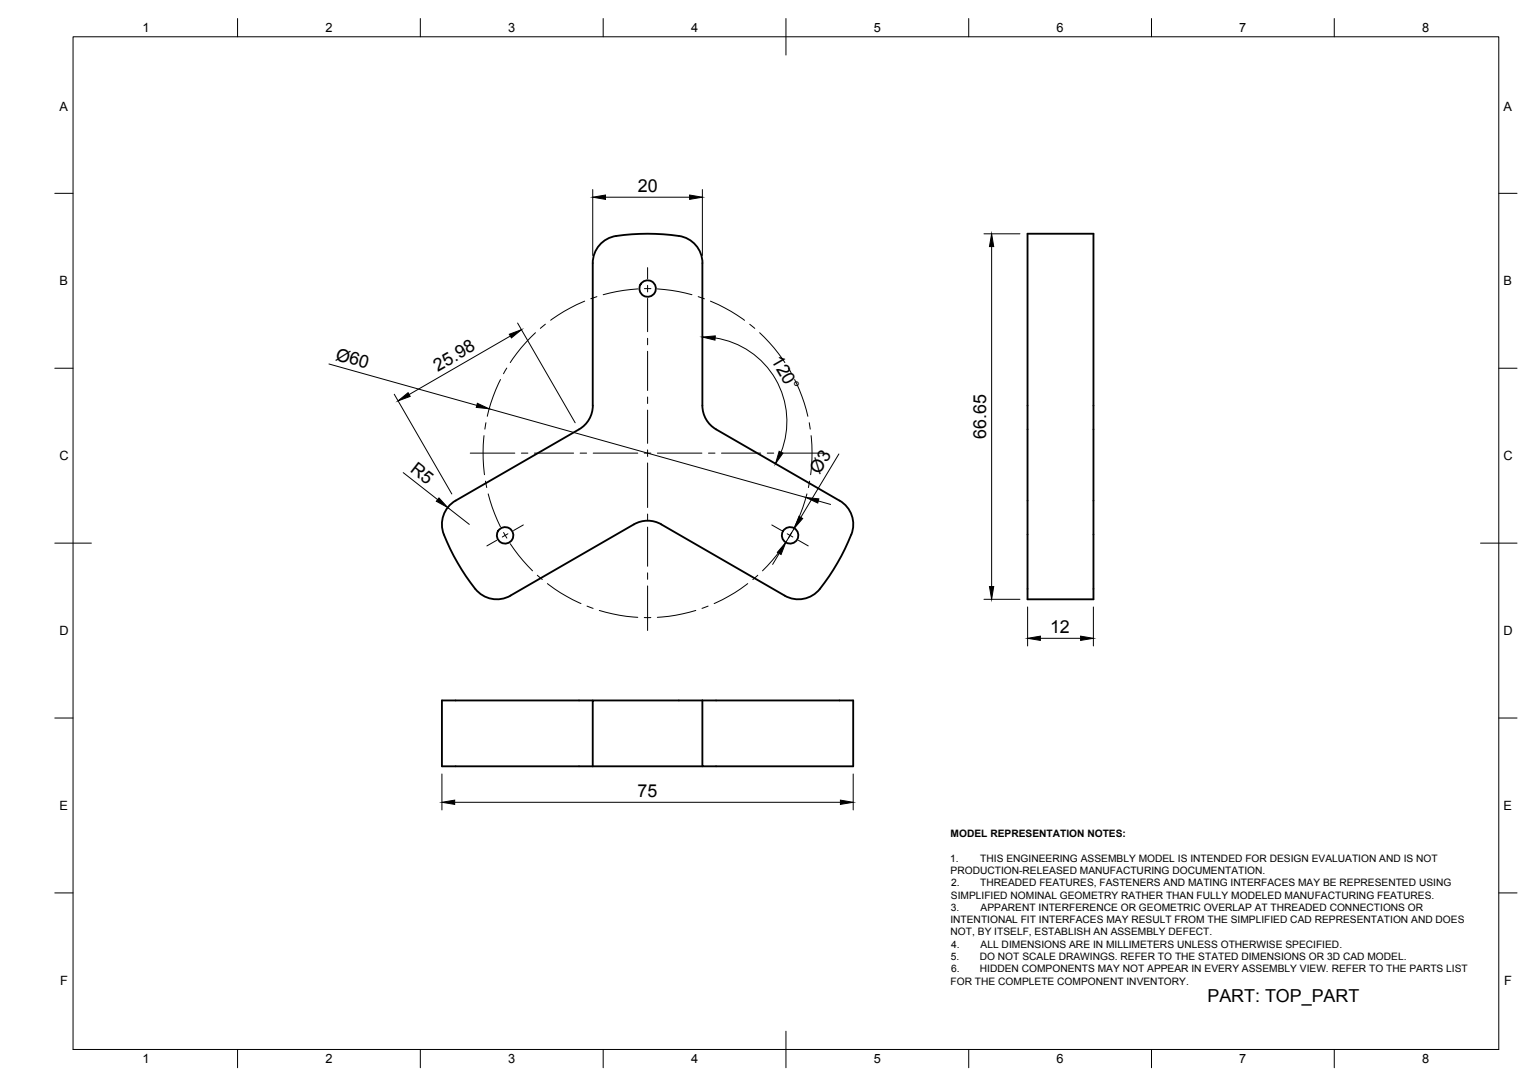
ISO-10303-21;
HEADER;
/* Generated by software containing ST-Developer
 * from STEP Tools, Inc. (www.steptools.com) 
 */

FILE_DESCRIPTION(
/* description */ (''),
/* implementation_level */ '2;1');

FILE_NAME(
/* name */ 'Top_Part.step',
/* time_stamp */ '2026-10-05T00:14:20-07:00',
/* author */ (''),
/* organization */ (''),
/* preprocessor_version */ 'ST-DEVELOPER v20.2',
/* originating_system */ 'Autodesk Translation Framework v15.15.0.0',
/* authorisation */ '');

FILE_SCHEMA (('AUTOMOTIVE_DESIGN { 1 0 10303 214 3 1 1 }'));
ENDSEC;

DATA;
#10=MECHANICAL_DESIGN_GEOMETRIC_PRESENTATION_REPRESENTATION('',(#3375),#75336);
#3359=SHAPE_REPRESENTATION_RELATIONSHIP('SRR','None',#75372,#3367);
#3367=ADVANCED_BREP_SHAPE_REPRESENTATION('',(#3383),#75332);
#3375=STYLED_ITEM('',(#75417),#3383);
#3383=MANIFOLD_SOLID_BREP('Body1',#32025);
#3388=FACE_BOUND('',#6889,.T.);
#3389=FACE_BOUND('',#6890,.T.);
#3390=FACE_BOUND('',#6891,.T.);
#3391=FACE_BOUND('',#6903,.T.);
#3392=FACE_BOUND('',#6904,.T.);
#3393=FACE_BOUND('',#6905,.T.);
#3405=CIRCLE('',#32145,1.5);
#3406=CIRCLE('',#32146,1.5);
#3407=CIRCLE('',#32148,1.5);
#3408=CIRCLE('',#32149,1.5);
#3409=CIRCLE('',#32151,1.5);
#3410=CIRCLE('',#32152,1.5);
#3411=CIRCLE('',#32154,5.);
#3412=CIRCLE('',#32155,5.);
#3413=CIRCLE('',#32158,5.);
#3414=CIRCLE('',#32159,5.);
#3415=CIRCLE('',#32162,5.);
#3416=CIRCLE('',#32163,5.);
#3417=CIRCLE('',#32166,5.);
#3418=CIRCLE('',#32167,5.);
#3419=CIRCLE('',#32169,40.);
#3420=CIRCLE('',#32170,40.);
#3421=CIRCLE('',#32172,5.);
#3422=CIRCLE('',#32173,40.);
#3423=CIRCLE('',#32174,5.);
#3424=CIRCLE('',#32175,5.);
#3425=CIRCLE('',#32176,40.);
#3426=CIRCLE('',#32177,5.);
#3427=CIRCLE('',#32178,5.);
#3428=CIRCLE('',#32180,5.);
#3429=CIRCLE('',#32182,40.);
#3430=CIRCLE('',#32184,5.);
#3431=CIRCLE('',#32186,5.);
#3432=CIRCLE('',#32188,5.);
#3433=CIRCLE('',#32190,5.);
#3434=CIRCLE('',#32193,40.);
#4456=CYLINDRICAL_SURFACE('',#32144,1.5);
#4457=CYLINDRICAL_SURFACE('',#32147,1.5);
#4458=CYLINDRICAL_SURFACE('',#32150,1.5);
#4459=CYLINDRICAL_SURFACE('',#32153,5.);
#4460=CYLINDRICAL_SURFACE('',#32157,5.);
#4461=CYLINDRICAL_SURFACE('',#32161,5.);
#4462=CYLINDRICAL_SURFACE('',#32165,5.);
#4463=CYLINDRICAL_SURFACE('',#32168,40.);
#4464=CYLINDRICAL_SURFACE('',#32179,5.);
#4465=CYLINDRICAL_SURFACE('',#32181,40.);
#4466=CYLINDRICAL_SURFACE('',#32183,5.);
#4467=CYLINDRICAL_SURFACE('',#32185,5.);
#4468=CYLINDRICAL_SURFACE('',#32187,5.);
#4469=CYLINDRICAL_SURFACE('',#32189,5.);
#4470=CYLINDRICAL_SURFACE('',#32192,40.);
#5149=FACE_OUTER_BOUND('',#6877,.T.);
#5150=FACE_OUTER_BOUND('',#6878,.T.);
#5151=FACE_OUTER_BOUND('',#6879,.T.);
#5152=FACE_OUTER_BOUND('',#6880,.T.);
#5153=FACE_OUTER_BOUND('',#6881,.T.);
#5154=FACE_OUTER_BOUND('',#6882,.T.);
#5155=FACE_OUTER_BOUND('',#6883,.T.);
#5156=FACE_OUTER_BOUND('',#6884,.T.);
#5157=FACE_OUTER_BOUND('',#6885,.T.);
#5158=FACE_OUTER_BOUND('',#6886,.T.);
#5159=FACE_OUTER_BOUND('',#6887,.T.);
#5160=FACE_OUTER_BOUND('',#6888,.T.);
#5161=FACE_OUTER_BOUND('',#6892,.T.);
#5162=FACE_OUTER_BOUND('',#6893,.T.);
#5163=FACE_OUTER_BOUND('',#6894,.T.);
#5164=FACE_OUTER_BOUND('',#6895,.T.);
#5165=FACE_OUTER_BOUND('',#6896,.T.);
#5166=FACE_OUTER_BOUND('',#6897,.T.);
#5167=FACE_OUTER_BOUND('',#6898,.T.);
#5168=FACE_OUTER_BOUND('',#6899,.T.);
#5169=FACE_OUTER_BOUND('',#6900,.T.);
#5170=FACE_OUTER_BOUND('',#6901,.T.);
#5171=FACE_OUTER_BOUND('',#6902,.T.);
#6877=EDGE_LOOP('',(#19631,#19632,#19633,#19634));
#6878=EDGE_LOOP('',(#19635,#19636,#19637,#19638));
#6879=EDGE_LOOP('',(#19639,#19640,#19641,#19642));
#6880=EDGE_LOOP('',(#19643,#19644,#19645,#19646));
#6881=EDGE_LOOP('',(#19647,#19648,#19649,#19650));
#6882=EDGE_LOOP('',(#19651,#19652,#19653,#19654));
#6883=EDGE_LOOP('',(#19655,#19656,#19657,#19658));
#6884=EDGE_LOOP('',(#19659,#19660,#19661,#19662));
#6885=EDGE_LOOP('',(#19663,#19664,#19665,#19666));
#6886=EDGE_LOOP('',(#19667,#19668,#19669,#19670));
#6887=EDGE_LOOP('',(#19671,#19672,#19673,#19674));
#6888=EDGE_LOOP('',(#19675,#19676,#19677,#19678,#19679,#19680,#19681,#19682,
#19683,#19684,#19685,#19686,#19687,#19688,#19689,#19690,#19691,#19692));
#6889=EDGE_LOOP('',(#19693));
#6890=EDGE_LOOP('',(#19694));
#6891=EDGE_LOOP('',(#19695));
#6892=EDGE_LOOP('',(#19696,#19697,#19698,#19699));
#6893=EDGE_LOOP('',(#19700,#19701,#19702,#19703));
#6894=EDGE_LOOP('',(#19704,#19705,#19706,#19707));
#6895=EDGE_LOOP('',(#19708,#19709,#19710,#19711));
#6896=EDGE_LOOP('',(#19712,#19713,#19714,#19715));
#6897=EDGE_LOOP('',(#19716,#19717,#19718,#19719));
#6898=EDGE_LOOP('',(#19720,#19721,#19722,#19723));
#6899=EDGE_LOOP('',(#19724,#19725,#19726,#19727));
#6900=EDGE_LOOP('',(#19728,#19729,#19730,#19731));
#6901=EDGE_LOOP('',(#19732,#19733,#19734,#19735));
#6902=EDGE_LOOP('',(#19736,#19737,#19738,#19739,#19740,#19741,#19742,#19743,
#19744,#19745,#19746,#19747,#19748,#19749,#19750,#19751,#19752,#19753));
#6903=EDGE_LOOP('',(#19754));
#6904=EDGE_LOOP('',(#19755));
#6905=EDGE_LOOP('',(#19756));
#8623=LINE('',#46118,#9869);
#8624=LINE('',#46124,#9870);
#8625=LINE('',#46130,#9871);
#8626=LINE('',#46137,#9872);
#8627=LINE('',#46140,#9873);
#8628=LINE('',#46143,#9874);
#8629=LINE('',#46145,#9875);
#8630=LINE('',#46146,#9876);
#8631=LINE('',#46152,#9877);
#8632=LINE('',#46155,#9878);
#8633=LINE('',#46158,#9879);
#8634=LINE('',#46160,#9880);
#8635=LINE('',#46161,#9881);
#8636=LINE('',#46167,#9882);
#8637=LINE('',#46170,#9883);
#8638=LINE('',#46173,#9884);
#8639=LINE('',#46175,#9885);
#8640=LINE('',#46176,#9886);
#8641=LINE('',#46182,#9887);
#8642=LINE('',#46185,#9888);
#8643=LINE('',#46190,#9889);
#8644=LINE('',#46193,#9890);
#8645=LINE('',#46200,#9891);
#8646=LINE('',#46207,#9892);
#8647=LINE('',#46212,#9893);
#8648=LINE('',#46216,#9894);
#8649=LINE('',#46220,#9895);
#8650=LINE('',#46224,#9896);
#8651=LINE('',#46229,#9897);
#8652=LINE('',#46232,#9898);
#8653=LINE('',#46234,#9899);
#8654=LINE('',#46238,#9900);
#8655=LINE('',#46240,#9901);
#9869=VECTOR('',#36423,1.5);
#9870=VECTOR('',#36430,1.5);
#9871=VECTOR('',#36437,1.5);
#9872=VECTOR('',#36444,10.);
#9873=VECTOR('',#36447,10.);
#9874=VECTOR('',#36450,10.);
#9875=VECTOR('',#36451,10.);
#9876=VECTOR('',#36452,10.);
#9877=VECTOR('',#36457,10.);
#9878=VECTOR('',#36460,10.);
#9879=VECTOR('',#36463,10.);
#9880=VECTOR('',#36464,10.);
#9881=VECTOR('',#36465,10.);
#9882=VECTOR('',#36470,10.);
#9883=VECTOR('',#36473,10.);
#9884=VECTOR('',#36476,9.99999999999999);
#9885=VECTOR('',#36477,10.);
#9886=VECTOR('',#36478,9.99999999999999);
#9887=VECTOR('',#36483,10.);
#9888=VECTOR('',#36486,10.);
#9889=VECTOR('',#36491,10.);
#9890=VECTOR('',#36496,9.99999999999999);
#9891=VECTOR('',#36503,10.);
#9892=VECTOR('',#36510,10.);
#9893=VECTOR('',#36517,10.);
#9894=VECTOR('',#36522,10.);
#9895=VECTOR('',#36527,10.);
#9896=VECTOR('',#36532,10.);
#9897=VECTOR('',#36539,10.);
#9898=VECTOR('',#36542,10.);
#9899=VECTOR('',#36545,10.);
#9900=VECTOR('',#36552,10.);
#9901=VECTOR('',#36555,9.99999999999999);
#11114=VERTEX_POINT('',#46115);
#11115=VERTEX_POINT('',#46117);
#11116=VERTEX_POINT('',#46121);
#11117=VERTEX_POINT('',#46123);
#11118=VERTEX_POINT('',#46127);
#11119=VERTEX_POINT('',#46129);
#11120=VERTEX_POINT('',#46133);
#11121=VERTEX_POINT('',#46134);
#11122=VERTEX_POINT('',#46136);
#11123=VERTEX_POINT('',#46138);
#11124=VERTEX_POINT('',#46142);
#11125=VERTEX_POINT('',#46144);
#11126=VERTEX_POINT('',#46148);
#11127=VERTEX_POINT('',#46149);
#11128=VERTEX_POINT('',#46151);
#11129=VERTEX_POINT('',#46153);
#11130=VERTEX_POINT('',#46157);
#11131=VERTEX_POINT('',#46159);
#11132=VERTEX_POINT('',#46163);
#11133=VERTEX_POINT('',#46164);
#11134=VERTEX_POINT('',#46166);
#11135=VERTEX_POINT('',#46168);
#11136=VERTEX_POINT('',#46172);
#11137=VERTEX_POINT('',#46174);
#11138=VERTEX_POINT('',#46178);
#11139=VERTEX_POINT('',#46179);
#11140=VERTEX_POINT('',#46181);
#11141=VERTEX_POINT('',#46183);
#11142=VERTEX_POINT('',#46187);
#11143=VERTEX_POINT('',#46189);
#11144=VERTEX_POINT('',#46194);
#11145=VERTEX_POINT('',#46196);
#11146=VERTEX_POINT('',#46198);
#11147=VERTEX_POINT('',#46201);
#11148=VERTEX_POINT('',#46203);
#11149=VERTEX_POINT('',#46205);
#11150=VERTEX_POINT('',#46210);
#11151=VERTEX_POINT('',#46214);
#11152=VERTEX_POINT('',#46218);
#11153=VERTEX_POINT('',#46222);
#11154=VERTEX_POINT('',#46228);
#11155=VERTEX_POINT('',#46230);
#14510=EDGE_CURVE('',#11114,#11114,#3405,.T.);
#14511=EDGE_CURVE('',#11114,#11115,#8623,.T.);
#14512=EDGE_CURVE('',#11115,#11115,#3406,.T.);
#14513=EDGE_CURVE('',#11116,#11116,#3407,.T.);
#14514=EDGE_CURVE('',#11116,#11117,#8624,.T.);
#14515=EDGE_CURVE('',#11117,#11117,#3408,.T.);
#14516=EDGE_CURVE('',#11118,#11118,#3409,.T.);
#14517=EDGE_CURVE('',#11118,#11119,#8625,.T.);
#14518=EDGE_CURVE('',#11119,#11119,#3410,.T.);
#14519=EDGE_CURVE('',#11120,#11121,#3411,.T.);
#14520=EDGE_CURVE('',#11121,#11122,#8626,.T.);
#14521=EDGE_CURVE('',#11122,#11123,#3412,.T.);
#14522=EDGE_CURVE('',#11123,#11120,#8627,.T.);
#14523=EDGE_CURVE('',#11121,#11124,#8628,.T.);
#14524=EDGE_CURVE('',#11125,#11124,#8629,.T.);
#14525=EDGE_CURVE('',#11122,#11125,#8630,.T.);
#14526=EDGE_CURVE('',#11126,#11127,#3413,.T.);
#14527=EDGE_CURVE('',#11127,#11128,#8631,.T.);
#14528=EDGE_CURVE('',#11128,#11129,#3414,.T.);
#14529=EDGE_CURVE('',#11129,#11126,#8632,.T.);
#14530=EDGE_CURVE('',#11127,#11130,#8633,.T.);
#14531=EDGE_CURVE('',#11131,#11130,#8634,.T.);
#14532=EDGE_CURVE('',#11128,#11131,#8635,.T.);
#14533=EDGE_CURVE('',#11132,#11133,#3415,.T.);
#14534=EDGE_CURVE('',#11133,#11134,#8636,.T.);
#14535=EDGE_CURVE('',#11134,#11135,#3416,.T.);
#14536=EDGE_CURVE('',#11135,#11132,#8637,.T.);
#14537=EDGE_CURVE('',#11133,#11136,#8638,.T.);
#14538=EDGE_CURVE('',#11137,#11136,#8639,.T.);
#14539=EDGE_CURVE('',#11134,#11137,#8640,.T.);
#14540=EDGE_CURVE('',#11138,#11139,#3417,.T.);
#14541=EDGE_CURVE('',#11139,#11140,#8641,.T.);
#14542=EDGE_CURVE('',#11140,#11141,#3418,.T.);
#14543=EDGE_CURVE('',#11141,#11138,#8642,.T.);
#14544=EDGE_CURVE('',#11142,#11139,#3419,.T.);
#14545=EDGE_CURVE('',#11143,#11142,#8643,.T.);
#14546=EDGE_CURVE('',#11143,#11140,#3420,.T.);
#14547=EDGE_CURVE('',#11138,#11129,#8644,.T.);
#14548=EDGE_CURVE('',#11144,#11131,#3421,.T.);
#14549=EDGE_CURVE('',#11144,#11145,#3422,.T.);
#14550=EDGE_CURVE('',#11146,#11145,#3423,.T.);
#14551=EDGE_CURVE('',#11146,#11123,#8645,.T.);
#14552=EDGE_CURVE('',#11147,#11125,#3424,.T.);
#14553=EDGE_CURVE('',#11147,#11148,#3425,.T.);
#14554=EDGE_CURVE('',#11149,#11148,#3426,.T.);
#14555=EDGE_CURVE('',#11149,#11135,#8646,.T.);
#14556=EDGE_CURVE('',#11142,#11137,#3427,.T.);
#14557=EDGE_CURVE('',#11130,#11150,#3428,.T.);
#14558=EDGE_CURVE('',#11150,#11144,#8647,.T.);
#14559=EDGE_CURVE('',#11150,#11151,#3429,.T.);
#14560=EDGE_CURVE('',#11145,#11151,#8648,.T.);
#14561=EDGE_CURVE('',#11151,#11152,#3430,.T.);
#14562=EDGE_CURVE('',#11152,#11146,#8649,.T.);
#14563=EDGE_CURVE('',#11124,#11153,#3431,.T.);
#14564=EDGE_CURVE('',#11153,#11147,#8650,.T.);
#14565=EDGE_CURVE('',#11136,#11143,#3432,.T.);
#14566=EDGE_CURVE('',#11148,#11154,#8651,.T.);
#14567=EDGE_CURVE('',#11154,#11155,#3433,.T.);
#14568=EDGE_CURVE('',#11155,#11149,#8652,.T.);
#14569=EDGE_CURVE('',#11155,#11132,#8653,.T.);
#14570=EDGE_CURVE('',#11153,#11154,#3434,.T.);
#14571=EDGE_CURVE('',#11152,#11120,#8654,.T.);
#14572=EDGE_CURVE('',#11141,#11126,#8655,.T.);
#19631=ORIENTED_EDGE('',*,*,#14510,.F.);
#19632=ORIENTED_EDGE('',*,*,#14511,.T.);
#19633=ORIENTED_EDGE('',*,*,#14512,.F.);
#19634=ORIENTED_EDGE('',*,*,#14511,.F.);
#19635=ORIENTED_EDGE('',*,*,#14513,.F.);
#19636=ORIENTED_EDGE('',*,*,#14514,.T.);
#19637=ORIENTED_EDGE('',*,*,#14515,.F.);
#19638=ORIENTED_EDGE('',*,*,#14514,.F.);
#19639=ORIENTED_EDGE('',*,*,#14516,.F.);
#19640=ORIENTED_EDGE('',*,*,#14517,.T.);
#19641=ORIENTED_EDGE('',*,*,#14518,.F.);
#19642=ORIENTED_EDGE('',*,*,#14517,.F.);
#19643=ORIENTED_EDGE('',*,*,#14519,.T.);
#19644=ORIENTED_EDGE('',*,*,#14520,.T.);
#19645=ORIENTED_EDGE('',*,*,#14521,.T.);
#19646=ORIENTED_EDGE('',*,*,#14522,.T.);
#19647=ORIENTED_EDGE('',*,*,#14520,.F.);
#19648=ORIENTED_EDGE('',*,*,#14523,.T.);
#19649=ORIENTED_EDGE('',*,*,#14524,.F.);
#19650=ORIENTED_EDGE('',*,*,#14525,.F.);
#19651=ORIENTED_EDGE('',*,*,#14526,.T.);
#19652=ORIENTED_EDGE('',*,*,#14527,.T.);
#19653=ORIENTED_EDGE('',*,*,#14528,.T.);
#19654=ORIENTED_EDGE('',*,*,#14529,.T.);
#19655=ORIENTED_EDGE('',*,*,#14527,.F.);
#19656=ORIENTED_EDGE('',*,*,#14530,.T.);
#19657=ORIENTED_EDGE('',*,*,#14531,.F.);
#19658=ORIENTED_EDGE('',*,*,#14532,.F.);
#19659=ORIENTED_EDGE('',*,*,#14533,.T.);
#19660=ORIENTED_EDGE('',*,*,#14534,.T.);
#19661=ORIENTED_EDGE('',*,*,#14535,.T.);
#19662=ORIENTED_EDGE('',*,*,#14536,.T.);
#19663=ORIENTED_EDGE('',*,*,#14534,.F.);
#19664=ORIENTED_EDGE('',*,*,#14537,.T.);
#19665=ORIENTED_EDGE('',*,*,#14538,.F.);
#19666=ORIENTED_EDGE('',*,*,#14539,.F.);
#19667=ORIENTED_EDGE('',*,*,#14540,.T.);
#19668=ORIENTED_EDGE('',*,*,#14541,.T.);
#19669=ORIENTED_EDGE('',*,*,#14542,.T.);
#19670=ORIENTED_EDGE('',*,*,#14543,.T.);
#19671=ORIENTED_EDGE('',*,*,#14541,.F.);
#19672=ORIENTED_EDGE('',*,*,#14544,.F.);
#19673=ORIENTED_EDGE('',*,*,#14545,.F.);
#19674=ORIENTED_EDGE('',*,*,#14546,.T.);
#19675=ORIENTED_EDGE('',*,*,#14540,.F.);
#19676=ORIENTED_EDGE('',*,*,#14547,.T.);
#19677=ORIENTED_EDGE('',*,*,#14528,.F.);
#19678=ORIENTED_EDGE('',*,*,#14532,.T.);
#19679=ORIENTED_EDGE('',*,*,#14548,.F.);
#19680=ORIENTED_EDGE('',*,*,#14549,.T.);
#19681=ORIENTED_EDGE('',*,*,#14550,.F.);
#19682=ORIENTED_EDGE('',*,*,#14551,.T.);
#19683=ORIENTED_EDGE('',*,*,#14521,.F.);
#19684=ORIENTED_EDGE('',*,*,#14525,.T.);
#19685=ORIENTED_EDGE('',*,*,#14552,.F.);
#19686=ORIENTED_EDGE('',*,*,#14553,.T.);
#19687=ORIENTED_EDGE('',*,*,#14554,.F.);
#19688=ORIENTED_EDGE('',*,*,#14555,.T.);
#19689=ORIENTED_EDGE('',*,*,#14535,.F.);
#19690=ORIENTED_EDGE('',*,*,#14539,.T.);
#19691=ORIENTED_EDGE('',*,*,#14556,.F.);
#19692=ORIENTED_EDGE('',*,*,#14544,.T.);
#19693=ORIENTED_EDGE('',*,*,#14510,.T.);
#19694=ORIENTED_EDGE('',*,*,#14513,.T.);
#19695=ORIENTED_EDGE('',*,*,#14516,.T.);
#19696=ORIENTED_EDGE('',*,*,#14548,.T.);
#19697=ORIENTED_EDGE('',*,*,#14531,.T.);
#19698=ORIENTED_EDGE('',*,*,#14557,.T.);
#19699=ORIENTED_EDGE('',*,*,#14558,.T.);
#19700=ORIENTED_EDGE('',*,*,#14558,.F.);
#19701=ORIENTED_EDGE('',*,*,#14559,.T.);
#19702=ORIENTED_EDGE('',*,*,#14560,.F.);
#19703=ORIENTED_EDGE('',*,*,#14549,.F.);
#19704=ORIENTED_EDGE('',*,*,#14550,.T.);
#19705=ORIENTED_EDGE('',*,*,#14560,.T.);
#19706=ORIENTED_EDGE('',*,*,#14561,.T.);
#19707=ORIENTED_EDGE('',*,*,#14562,.T.);
#19708=ORIENTED_EDGE('',*,*,#14552,.T.);
#19709=ORIENTED_EDGE('',*,*,#14524,.T.);
#19710=ORIENTED_EDGE('',*,*,#14563,.T.);
#19711=ORIENTED_EDGE('',*,*,#14564,.T.);
#19712=ORIENTED_EDGE('',*,*,#14556,.T.);
#19713=ORIENTED_EDGE('',*,*,#14538,.T.);
#19714=ORIENTED_EDGE('',*,*,#14565,.T.);
#19715=ORIENTED_EDGE('',*,*,#14545,.T.);
#19716=ORIENTED_EDGE('',*,*,#14554,.T.);
#19717=ORIENTED_EDGE('',*,*,#14566,.T.);
#19718=ORIENTED_EDGE('',*,*,#14567,.T.);
#19719=ORIENTED_EDGE('',*,*,#14568,.T.);
#19720=ORIENTED_EDGE('',*,*,#14536,.F.);
#19721=ORIENTED_EDGE('',*,*,#14555,.F.);
#19722=ORIENTED_EDGE('',*,*,#14568,.F.);
#19723=ORIENTED_EDGE('',*,*,#14569,.T.);
#19724=ORIENTED_EDGE('',*,*,#14564,.F.);
#19725=ORIENTED_EDGE('',*,*,#14570,.T.);
#19726=ORIENTED_EDGE('',*,*,#14566,.F.);
#19727=ORIENTED_EDGE('',*,*,#14553,.F.);
#19728=ORIENTED_EDGE('',*,*,#14522,.F.);
#19729=ORIENTED_EDGE('',*,*,#14551,.F.);
#19730=ORIENTED_EDGE('',*,*,#14562,.F.);
#19731=ORIENTED_EDGE('',*,*,#14571,.T.);
#19732=ORIENTED_EDGE('',*,*,#14529,.F.);
#19733=ORIENTED_EDGE('',*,*,#14547,.F.);
#19734=ORIENTED_EDGE('',*,*,#14543,.F.);
#19735=ORIENTED_EDGE('',*,*,#14572,.T.);
#19736=ORIENTED_EDGE('',*,*,#14542,.F.);
#19737=ORIENTED_EDGE('',*,*,#14546,.F.);
#19738=ORIENTED_EDGE('',*,*,#14565,.F.);
#19739=ORIENTED_EDGE('',*,*,#14537,.F.);
#19740=ORIENTED_EDGE('',*,*,#14533,.F.);
#19741=ORIENTED_EDGE('',*,*,#14569,.F.);
#19742=ORIENTED_EDGE('',*,*,#14567,.F.);
#19743=ORIENTED_EDGE('',*,*,#14570,.F.);
#19744=ORIENTED_EDGE('',*,*,#14563,.F.);
#19745=ORIENTED_EDGE('',*,*,#14523,.F.);
#19746=ORIENTED_EDGE('',*,*,#14519,.F.);
#19747=ORIENTED_EDGE('',*,*,#14571,.F.);
#19748=ORIENTED_EDGE('',*,*,#14561,.F.);
#19749=ORIENTED_EDGE('',*,*,#14559,.F.);
#19750=ORIENTED_EDGE('',*,*,#14557,.F.);
#19751=ORIENTED_EDGE('',*,*,#14530,.F.);
#19752=ORIENTED_EDGE('',*,*,#14526,.F.);
#19753=ORIENTED_EDGE('',*,*,#14572,.F.);
#19754=ORIENTED_EDGE('',*,*,#14512,.T.);
#19755=ORIENTED_EDGE('',*,*,#14515,.T.);
#19756=ORIENTED_EDGE('',*,*,#14518,.T.);
#29776=PLANE('',#32156);
#29777=PLANE('',#32160);
#29778=PLANE('',#32164);
#29779=PLANE('',#32171);
#29780=PLANE('',#32191);
#29781=PLANE('',#32194);
#29782=PLANE('',#32195);
#29783=PLANE('',#32196);
#30309=ADVANCED_FACE('',(#5149),#4456,.F.);
#30310=ADVANCED_FACE('',(#5150),#4457,.F.);
#30311=ADVANCED_FACE('',(#5151),#4458,.F.);
#30312=ADVANCED_FACE('',(#5152),#4459,.F.);
#30313=ADVANCED_FACE('',(#5153),#29776,.T.);
#30314=ADVANCED_FACE('',(#5154),#4460,.F.);
#30315=ADVANCED_FACE('',(#5155),#29777,.T.);
#30316=ADVANCED_FACE('',(#5156),#4461,.F.);
#30317=ADVANCED_FACE('',(#5157),#29778,.T.);
#30318=ADVANCED_FACE('',(#5158),#4462,.T.);
#30319=ADVANCED_FACE('',(#5159),#4463,.T.);
#30320=ADVANCED_FACE('',(#5160,#3388,#3389,#3390),#29779,.T.);
#30321=ADVANCED_FACE('',(#5161),#4464,.T.);
#30322=ADVANCED_FACE('',(#5162),#4465,.T.);
#30323=ADVANCED_FACE('',(#5163),#4466,.T.);
#30324=ADVANCED_FACE('',(#5164),#4467,.T.);
#30325=ADVANCED_FACE('',(#5165),#4468,.T.);
#30326=ADVANCED_FACE('',(#5166),#4469,.T.);
#30327=ADVANCED_FACE('',(#5167),#29780,.T.);
#30328=ADVANCED_FACE('',(#5168),#4470,.T.);
#30329=ADVANCED_FACE('',(#5169),#29781,.T.);
#30330=ADVANCED_FACE('',(#5170),#29782,.T.);
#30331=ADVANCED_FACE('',(#5171,#3391,#3392,#3393),#29783,.F.);
#32025=CLOSED_SHELL('',(#30309,#30310,#30311,#30312,#30313,#30314,#30315,
#30316,#30317,#30318,#30319,#30320,#30321,#30322,#30323,#30324,#30325,#30326,
#30327,#30328,#30329,#30330,#30331));
#32143=AXIS2_PLACEMENT_3D('',#46113,#36417,#36418);
#32144=AXIS2_PLACEMENT_3D('',#46114,#36419,#36420);
#32145=AXIS2_PLACEMENT_3D('',#46116,#36421,#36422);
#32146=AXIS2_PLACEMENT_3D('',#46119,#36424,#36425);
#32147=AXIS2_PLACEMENT_3D('',#46120,#36426,#36427);
#32148=AXIS2_PLACEMENT_3D('',#46122,#36428,#36429);
#32149=AXIS2_PLACEMENT_3D('',#46125,#36431,#36432);
#32150=AXIS2_PLACEMENT_3D('',#46126,#36433,#36434);
#32151=AXIS2_PLACEMENT_3D('',#46128,#36435,#36436);
#32152=AXIS2_PLACEMENT_3D('',#46131,#36438,#36439);
#32153=AXIS2_PLACEMENT_3D('',#46132,#36440,#36441);
#32154=AXIS2_PLACEMENT_3D('',#46135,#36442,#36443);
#32155=AXIS2_PLACEMENT_3D('',#46139,#36445,#36446);
#32156=AXIS2_PLACEMENT_3D('',#46141,#36448,#36449);
#32157=AXIS2_PLACEMENT_3D('',#46147,#36453,#36454);
#32158=AXIS2_PLACEMENT_3D('',#46150,#36455,#36456);
#32159=AXIS2_PLACEMENT_3D('',#46154,#36458,#36459);
#32160=AXIS2_PLACEMENT_3D('',#46156,#36461,#36462);
#32161=AXIS2_PLACEMENT_3D('',#46162,#36466,#36467);
#32162=AXIS2_PLACEMENT_3D('',#46165,#36468,#36469);
#32163=AXIS2_PLACEMENT_3D('',#46169,#36471,#36472);
#32164=AXIS2_PLACEMENT_3D('',#46171,#36474,#36475);
#32165=AXIS2_PLACEMENT_3D('',#46177,#36479,#36480);
#32166=AXIS2_PLACEMENT_3D('',#46180,#36481,#36482);
#32167=AXIS2_PLACEMENT_3D('',#46184,#36484,#36485);
#32168=AXIS2_PLACEMENT_3D('',#46186,#36487,#36488);
#32169=AXIS2_PLACEMENT_3D('',#46188,#36489,#36490);
#32170=AXIS2_PLACEMENT_3D('',#46191,#36492,#36493);
#32171=AXIS2_PLACEMENT_3D('',#46192,#36494,#36495);
#32172=AXIS2_PLACEMENT_3D('',#46195,#36497,#36498);
#32173=AXIS2_PLACEMENT_3D('',#46197,#36499,#36500);
#32174=AXIS2_PLACEMENT_3D('',#46199,#36501,#36502);
#32175=AXIS2_PLACEMENT_3D('',#46202,#36504,#36505);
#32176=AXIS2_PLACEMENT_3D('',#46204,#36506,#36507);
#32177=AXIS2_PLACEMENT_3D('',#46206,#36508,#36509);
#32178=AXIS2_PLACEMENT_3D('',#46208,#36511,#36512);
#32179=AXIS2_PLACEMENT_3D('',#46209,#36513,#36514);
#32180=AXIS2_PLACEMENT_3D('',#46211,#36515,#36516);
#32181=AXIS2_PLACEMENT_3D('',#46213,#36518,#36519);
#32182=AXIS2_PLACEMENT_3D('',#46215,#36520,#36521);
#32183=AXIS2_PLACEMENT_3D('',#46217,#36523,#36524);
#32184=AXIS2_PLACEMENT_3D('',#46219,#36525,#36526);
#32185=AXIS2_PLACEMENT_3D('',#46221,#36528,#36529);
#32186=AXIS2_PLACEMENT_3D('',#46223,#36530,#36531);
#32187=AXIS2_PLACEMENT_3D('',#46225,#36533,#36534);
#32188=AXIS2_PLACEMENT_3D('',#46226,#36535,#36536);
#32189=AXIS2_PLACEMENT_3D('',#46227,#36537,#36538);
#32190=AXIS2_PLACEMENT_3D('',#46231,#36540,#36541);
#32191=AXIS2_PLACEMENT_3D('',#46233,#36543,#36544);
#32192=AXIS2_PLACEMENT_3D('',#46235,#36546,#36547);
#32193=AXIS2_PLACEMENT_3D('',#46236,#36548,#36549);
#32194=AXIS2_PLACEMENT_3D('',#46237,#36550,#36551);
#32195=AXIS2_PLACEMENT_3D('',#46239,#36553,#36554);
#32196=AXIS2_PLACEMENT_3D('',#46241,#36556,#36557);
#36417=DIRECTION('axis',(0.,0.,1.));
#36418=DIRECTION('refdir',(1.,0.,0.));
#36419=DIRECTION('center_axis',(0.,0.,-1.));
#36420=DIRECTION('ref_axis',(0.5,0.866025403784438,0.));
#36421=DIRECTION('center_axis',(0.,0.,-1.));
#36422=DIRECTION('ref_axis',(0.5,0.866025403784438,0.));
#36423=DIRECTION('',(0.,0.,-1.));
#36424=DIRECTION('center_axis',(0.,0.,1.));
#36425=DIRECTION('ref_axis',(0.5,0.866025403784438,0.));
#36426=DIRECTION('center_axis',(0.,0.,-1.));
#36427=DIRECTION('ref_axis',(0.5,-0.866025403784439,0.));
#36428=DIRECTION('center_axis',(0.,0.,-1.));
#36429=DIRECTION('ref_axis',(0.5,-0.866025403784439,0.));
#36430=DIRECTION('',(0.,0.,-1.));
#36431=DIRECTION('center_axis',(0.,0.,1.));
#36432=DIRECTION('ref_axis',(0.5,-0.866025403784439,0.));
#36433=DIRECTION('center_axis',(0.,0.,-1.));
#36434=DIRECTION('ref_axis',(-1.,0.,0.));
#36435=DIRECTION('center_axis',(0.,0.,-1.));
#36436=DIRECTION('ref_axis',(-1.,0.,0.));
#36437=DIRECTION('',(0.,0.,-1.));
#36438=DIRECTION('center_axis',(0.,0.,1.));
#36439=DIRECTION('ref_axis',(-1.,0.,0.));
#36440=DIRECTION('center_axis',(0.,0.,1.));
#36441=DIRECTION('ref_axis',(-0.5,-0.866025403784439,0.));
#36442=DIRECTION('center_axis',(0.,0.,-1.));
#36443=DIRECTION('ref_axis',(-0.5,-0.866025403784439,0.));
#36444=DIRECTION('',(0.,0.,1.));
#36445=DIRECTION('center_axis',(0.,0.,1.));
#36446=DIRECTION('ref_axis',(-0.5,-0.866025403784439,0.));
#36447=DIRECTION('',(0.,0.,-1.));
#36448=DIRECTION('center_axis',(0.866025403784439,0.5,0.));
#36449=DIRECTION('ref_axis',(-0.5,0.866025403784439,0.));
#36450=DIRECTION('',(-0.5,0.866025403784439,0.));
#36451=DIRECTION('',(0.,0.,-1.));
#36452=DIRECTION('',(-0.5,0.866025403784439,0.));
#36453=DIRECTION('center_axis',(0.,0.,1.));
#36454=DIRECTION('ref_axis',(-0.5,0.866025403784439,0.));
#36455=DIRECTION('center_axis',(0.,0.,-1.));
#36456=DIRECTION('ref_axis',(-0.5,0.866025403784439,0.));
#36457=DIRECTION('',(0.,0.,1.));
#36458=DIRECTION('center_axis',(0.,0.,1.));
#36459=DIRECTION('ref_axis',(-0.5,0.866025403784439,0.));
#36460=DIRECTION('',(0.,0.,-1.));
#36461=DIRECTION('center_axis',(0.,-1.,0.));
#36462=DIRECTION('ref_axis',(1.,0.,0.));
#36463=DIRECTION('',(1.,0.,0.));
#36464=DIRECTION('',(0.,0.,-1.));
#36465=DIRECTION('',(1.,0.,0.));
#36466=DIRECTION('center_axis',(0.,0.,1.));
#36467=DIRECTION('ref_axis',(1.,-1.92296268638356E-16,0.));
#36468=DIRECTION('center_axis',(0.,0.,-1.));
#36469=DIRECTION('ref_axis',(1.,-1.92296268638356E-16,0.));
#36470=DIRECTION('',(0.,0.,1.));
#36471=DIRECTION('center_axis',(0.,0.,1.));
#36472=DIRECTION('ref_axis',(1.,-1.92296268638356E-16,0.));
#36473=DIRECTION('',(0.,0.,-1.));
#36474=DIRECTION('center_axis',(-0.866025403784438,0.5,0.));
#36475=DIRECTION('ref_axis',(-0.5,-0.866025403784438,0.));
#36476=DIRECTION('',(-0.5,-0.866025403784439,0.));
#36477=DIRECTION('',(0.,0.,-1.));
#36478=DIRECTION('',(-0.5,-0.866025403784439,0.));
#36479=DIRECTION('center_axis',(0.,0.,1.));
#36480=DIRECTION('ref_axis',(0.327326835353988,-0.944911182523068,0.));
#36481=DIRECTION('center_axis',(0.,0.,-1.));
#36482=DIRECTION('ref_axis',(0.327326835353988,-0.944911182523068,0.));
#36483=DIRECTION('',(0.,0.,-1.));
#36484=DIRECTION('center_axis',(0.,0.,1.));
#36485=DIRECTION('ref_axis',(0.327326835353988,-0.944911182523068,0.));
#36486=DIRECTION('',(0.,0.,1.));
#36487=DIRECTION('center_axis',(0.,0.,1.));
#36488=DIRECTION('ref_axis',(-1.,0.,0.));
#36489=DIRECTION('center_axis',(0.,0.,1.));
#36490=DIRECTION('ref_axis',(-1.,0.,0.));
#36491=DIRECTION('',(0.,0.,1.));
#36492=DIRECTION('center_axis',(0.,0.,1.));
#36493=DIRECTION('ref_axis',(-1.,0.,0.));
#36494=DIRECTION('center_axis',(0.,0.,1.));
#36495=DIRECTION('ref_axis',(-1.,0.,0.));
#36496=DIRECTION('',(0.5,0.866025403784439,0.));
#36497=DIRECTION('center_axis',(0.,0.,-1.));
#36498=DIRECTION('ref_axis',(0.654653670707978,-0.755928946018454,0.));
#36499=DIRECTION('center_axis',(0.,0.,1.));
#36500=DIRECTION('ref_axis',(-1.,0.,0.));
#36501=DIRECTION('center_axis',(0.,0.,-1.));
#36502=DIRECTION('ref_axis',(0.654653670707978,0.755928946018454,0.));
#36503=DIRECTION('',(-1.,0.,0.));
#36504=DIRECTION('center_axis',(0.,0.,-1.));
#36505=DIRECTION('ref_axis',(0.327326835353989,0.944911182523068,0.));
#36506=DIRECTION('center_axis',(0.,0.,1.));
#36507=DIRECTION('ref_axis',(-1.,0.,0.));
#36508=DIRECTION('center_axis',(0.,0.,-1.));
#36509=DIRECTION('ref_axis',(-0.981980506061966,0.188982236504613,0.));
#36510=DIRECTION('',(0.5,-0.866025403784439,0.));
#36511=DIRECTION('center_axis',(0.,0.,-1.));
#36512=DIRECTION('ref_axis',(-0.981980506061966,-0.188982236504613,0.));
#36513=DIRECTION('center_axis',(0.,0.,1.));
#36514=DIRECTION('ref_axis',(0.654653670707978,-0.755928946018454,0.));
#36515=DIRECTION('center_axis',(0.,0.,1.));
#36516=DIRECTION('ref_axis',(0.654653670707978,-0.755928946018454,0.));
#36517=DIRECTION('',(0.,0.,1.));
#36518=DIRECTION('center_axis',(0.,0.,1.));
#36519=DIRECTION('ref_axis',(1.,-1.22464679914735E-16,0.));
#36520=DIRECTION('center_axis',(0.,0.,1.));
#36521=DIRECTION('ref_axis',(-1.,0.,0.));
#36522=DIRECTION('',(0.,0.,-1.));
#36523=DIRECTION('center_axis',(0.,0.,1.));
#36524=DIRECTION('ref_axis',(0.654653670707978,0.755928946018454,0.));
#36525=DIRECTION('center_axis',(0.,0.,1.));
#36526=DIRECTION('ref_axis',(0.654653670707978,0.755928946018454,0.));
#36527=DIRECTION('',(0.,0.,1.));
#36528=DIRECTION('center_axis',(0.,0.,1.));
#36529=DIRECTION('ref_axis',(0.327326835353989,0.944911182523068,0.));
#36530=DIRECTION('center_axis',(0.,0.,1.));
#36531=DIRECTION('ref_axis',(0.327326835353989,0.944911182523068,0.));
#36532=DIRECTION('',(0.,0.,1.));
#36533=DIRECTION('center_axis',(0.,0.,1.));
#36534=DIRECTION('ref_axis',(-0.981980506061966,-0.188982236504613,0.));
#36535=DIRECTION('center_axis',(0.,0.,1.));
#36536=DIRECTION('ref_axis',(-0.981980506061966,-0.188982236504613,0.));
#36537=DIRECTION('center_axis',(0.,0.,1.));
#36538=DIRECTION('ref_axis',(-0.981980506061966,0.188982236504613,0.));
#36539=DIRECTION('',(0.,0.,-1.));
#36540=DIRECTION('center_axis',(0.,0.,1.));
#36541=DIRECTION('ref_axis',(-0.981980506061966,0.188982236504613,0.));
#36542=DIRECTION('',(0.,0.,1.));
#36543=DIRECTION('center_axis',(-0.866025403784439,-0.5,0.));
#36544=DIRECTION('ref_axis',(0.5,-0.866025403784439,0.));
#36545=DIRECTION('',(0.5,-0.866025403784439,0.));
#36546=DIRECTION('center_axis',(0.,0.,1.));
#36547=DIRECTION('ref_axis',(-1.,0.,0.));
#36548=DIRECTION('center_axis',(0.,0.,1.));
#36549=DIRECTION('ref_axis',(-1.,0.,0.));
#36550=DIRECTION('center_axis',(0.,1.,0.));
#36551=DIRECTION('ref_axis',(-1.,0.,0.));
#36552=DIRECTION('',(-1.,0.,0.));
#36553=DIRECTION('center_axis',(0.866025403784438,-0.5,0.));
#36554=DIRECTION('ref_axis',(0.5,0.866025403784438,0.));
#36555=DIRECTION('',(0.5,0.866025403784439,0.));
#36556=DIRECTION('center_axis',(0.,0.,1.));
#36557=DIRECTION('ref_axis',(-1.,0.,0.));
#46113=CARTESIAN_POINT('',(0.,0.,0.));
#46114=CARTESIAN_POINT('Origin',(-15.,-25.9807621135332,31.));
#46115=CARTESIAN_POINT('',(-15.75,-27.2798002192098,31.));
#46116=CARTESIAN_POINT('Origin',(-15.,-25.9807621135332,31.));
#46117=CARTESIAN_POINT('',(-15.75,-27.2798002192098,19.));
#46118=CARTESIAN_POINT('',(-15.75,-27.2798002192099,31.));
#46119=CARTESIAN_POINT('Origin',(-15.,-25.9807621135332,19.));
#46120=CARTESIAN_POINT('Origin',(-15.,25.9807621135332,31.));
#46121=CARTESIAN_POINT('',(-15.75,27.2798002192098,31.));
#46122=CARTESIAN_POINT('Origin',(-15.,25.9807621135332,31.));
#46123=CARTESIAN_POINT('',(-15.75,27.2798002192098,19.));
#46124=CARTESIAN_POINT('',(-15.75,27.2798002192099,31.));
#46125=CARTESIAN_POINT('Origin',(-15.,25.9807621135332,19.));
#46126=CARTESIAN_POINT('Origin',(30.,-9.99200722162641E-15,31.));
#46127=CARTESIAN_POINT('',(31.5,-9.8083102017543E-15,31.));
#46128=CARTESIAN_POINT('Origin',(30.,-9.99200722162641E-15,31.));
#46129=CARTESIAN_POINT('',(31.5,-9.8083102017543E-15,19.));
#46130=CARTESIAN_POINT('',(31.5,-1.01757042414985E-14,31.));
#46131=CARTESIAN_POINT('Origin',(30.,-9.99200722162641E-15,19.));
#46132=CARTESIAN_POINT('Origin',(8.66025403784439,15.,19.));
#46133=CARTESIAN_POINT('',(8.66025403784439,10.,19.));
#46134=CARTESIAN_POINT('',(4.3301270189222,12.5,19.));
#46135=CARTESIAN_POINT('Origin',(8.66025403784439,15.,19.));
#46136=CARTESIAN_POINT('',(4.3301270189222,12.5,31.));
#46137=CARTESIAN_POINT('',(4.3301270189222,12.5,19.));
#46138=CARTESIAN_POINT('',(8.66025403784439,10.,31.));
#46139=CARTESIAN_POINT('Origin',(8.66025403784439,15.,31.));
#46140=CARTESIAN_POINT('',(8.66025403784439,10.,19.));
#46141=CARTESIAN_POINT('Origin',(5.77350269189626,10.,19.));
#46142=CARTESIAN_POINT('',(-8.66025403784437,35.,19.));
#46143=CARTESIAN_POINT('',(8.66025403784439,5.,19.));
#46144=CARTESIAN_POINT('',(-8.66025403784437,35.,31.));
#46145=CARTESIAN_POINT('',(-8.66025403784438,35.,19.));
#46146=CARTESIAN_POINT('',(8.66025403784439,5.,31.));
#46147=CARTESIAN_POINT('Origin',(8.66025403784438,-15.,19.));
#46148=CARTESIAN_POINT('',(4.33012701892219,-12.5,19.));
#46149=CARTESIAN_POINT('',(8.66025403784438,-10.,19.));
#46150=CARTESIAN_POINT('Origin',(8.66025403784438,-15.,19.));
#46151=CARTESIAN_POINT('',(8.66025403784438,-10.,31.));
#46152=CARTESIAN_POINT('',(8.66025403784438,-10.,19.));
#46153=CARTESIAN_POINT('',(4.33012701892219,-12.5,31.));
#46154=CARTESIAN_POINT('Origin',(8.66025403784438,-15.,31.));
#46155=CARTESIAN_POINT('',(4.33012701892219,-12.5,19.));
#46156=CARTESIAN_POINT('Origin',(5.77350269189626,-10.,19.));
#46157=CARTESIAN_POINT('',(34.6410161513775,-10.,19.));
#46158=CARTESIAN_POINT('',(0.,-10.,19.));
#46159=CARTESIAN_POINT('',(34.6410161513775,-10.,31.));
#46160=CARTESIAN_POINT('',(34.6410161513775,-10.,19.));
#46161=CARTESIAN_POINT('',(0.,-10.,31.));
#46162=CARTESIAN_POINT('Origin',(-17.3205080756888,-2.22044604925031E-15,
19.));
#46163=CARTESIAN_POINT('',(-12.9903810567666,2.5,19.));
#46164=CARTESIAN_POINT('',(-12.9903810567666,-2.5,19.));
#46165=CARTESIAN_POINT('Origin',(-17.3205080756888,-2.22044604925031E-15,
19.));
#46166=CARTESIAN_POINT('',(-12.9903810567666,-2.5,31.));
#46167=CARTESIAN_POINT('',(-12.9903810567666,-2.5,19.));
#46168=CARTESIAN_POINT('',(-12.9903810567666,2.5,31.));
#46169=CARTESIAN_POINT('Origin',(-17.3205080756888,-2.22044604925031E-15,
31.));
#46170=CARTESIAN_POINT('',(-12.9903810567666,2.5,19.));
#46171=CARTESIAN_POINT('Origin',(-11.5470053837925,1.11022302462516E-15,
19.));
#46172=CARTESIAN_POINT('',(-25.9807621135332,-25.,19.));
#46173=CARTESIAN_POINT('',(-8.66025403784438,5.,19.));
#46174=CARTESIAN_POINT('',(-25.9807621135332,-25.,31.));
#46175=CARTESIAN_POINT('',(-25.9807621135332,-25.,19.));
#46176=CARTESIAN_POINT('',(-8.66025403784438,5.,31.));
#46177=CARTESIAN_POINT('Origin',(-12.9903810567666,-32.5,19.));
#46178=CARTESIAN_POINT('',(-8.6602540378444,-35.,31.));
#46179=CARTESIAN_POINT('',(-14.8461497791618,-37.1428571428571,31.));
#46180=CARTESIAN_POINT('Origin',(-12.9903810567666,-32.5,31.));
#46181=CARTESIAN_POINT('',(-14.8461497791618,-37.1428571428571,19.));
#46182=CARTESIAN_POINT('',(-14.8461497791618,-37.1428571428571,19.));
#46183=CARTESIAN_POINT('',(-8.6602540378444,-35.,19.));
#46184=CARTESIAN_POINT('Origin',(-12.9903810567666,-32.5,19.));
#46185=CARTESIAN_POINT('',(-8.6602540378444,-35.,19.));
#46186=CARTESIAN_POINT('Origin',(0.,0.,19.));
#46187=CARTESIAN_POINT('',(-24.7435829652697,-31.4285714285714,31.));
#46188=CARTESIAN_POINT('Origin',(0.,0.,31.));
#46189=CARTESIAN_POINT('',(-24.7435829652697,-31.4285714285714,19.));
#46190=CARTESIAN_POINT('',(-24.7435829652697,-31.4285714285714,19.));
#46191=CARTESIAN_POINT('Origin',(0.,0.,19.));
#46192=CARTESIAN_POINT('Origin',(5.98741461555926,0.,31.));
#46193=CARTESIAN_POINT('',(-10.7046626931927,-38.5410196624968,31.));
#46194=CARTESIAN_POINT('',(39.5897327444315,-5.71428571428572,31.));
#46195=CARTESIAN_POINT('Origin',(34.6410161513775,-5.,31.));
#46196=CARTESIAN_POINT('',(39.5897327444315,5.71428571428572,31.));
#46197=CARTESIAN_POINT('Origin',(0.,0.,31.));
#46198=CARTESIAN_POINT('',(34.6410161513775,10.,31.));
#46199=CARTESIAN_POINT('Origin',(34.6410161513775,5.,31.));
#46200=CARTESIAN_POINT('',(38.7298334620742,10.,31.));
#46201=CARTESIAN_POINT('',(-14.8461497791618,37.1428571428571,31.));
#46202=CARTESIAN_POINT('Origin',(-12.9903810567666,32.5,31.));
#46203=CARTESIAN_POINT('',(-24.7435829652697,31.4285714285714,31.));
#46204=CARTESIAN_POINT('Origin',(0.,0.,31.));
#46205=CARTESIAN_POINT('',(-25.9807621135332,25.,31.));
#46206=CARTESIAN_POINT('Origin',(-21.650635094611,27.5,31.));
#46207=CARTESIAN_POINT('',(-28.0251707688815,28.5410196624969,31.));
#46208=CARTESIAN_POINT('Origin',(-21.650635094611,-27.5,31.));
#46209=CARTESIAN_POINT('Origin',(34.6410161513775,-5.,19.));
#46210=CARTESIAN_POINT('',(39.5897327444315,-5.71428571428572,19.));
#46211=CARTESIAN_POINT('Origin',(34.6410161513775,-5.,19.));
#46212=CARTESIAN_POINT('',(39.5897327444315,-5.71428571428572,19.));
#46213=CARTESIAN_POINT('Origin',(0.,0.,19.));
#46214=CARTESIAN_POINT('',(39.5897327444315,5.71428571428572,19.));
#46215=CARTESIAN_POINT('Origin',(0.,0.,19.));
#46216=CARTESIAN_POINT('',(39.5897327444315,5.71428571428572,19.));
#46217=CARTESIAN_POINT('Origin',(34.6410161513775,5.,19.));
#46218=CARTESIAN_POINT('',(34.6410161513775,10.,19.));
#46219=CARTESIAN_POINT('Origin',(34.6410161513775,5.,19.));
#46220=CARTESIAN_POINT('',(34.6410161513775,10.,19.));
#46221=CARTESIAN_POINT('Origin',(-12.9903810567666,32.5,19.));
#46222=CARTESIAN_POINT('',(-14.8461497791618,37.1428571428571,19.));
#46223=CARTESIAN_POINT('Origin',(-12.9903810567666,32.5,19.));
#46224=CARTESIAN_POINT('',(-14.8461497791618,37.1428571428571,19.));
#46225=CARTESIAN_POINT('Origin',(-21.650635094611,-27.5,19.));
#46226=CARTESIAN_POINT('Origin',(-21.650635094611,-27.5,19.));
#46227=CARTESIAN_POINT('Origin',(-21.650635094611,27.5,19.));
#46228=CARTESIAN_POINT('',(-24.7435829652697,31.4285714285714,19.));
#46229=CARTESIAN_POINT('',(-24.7435829652697,31.4285714285714,19.));
#46230=CARTESIAN_POINT('',(-25.9807621135332,25.,19.));
#46231=CARTESIAN_POINT('Origin',(-21.650635094611,27.5,19.));
#46232=CARTESIAN_POINT('',(-25.9807621135332,25.,19.));
#46233=CARTESIAN_POINT('Origin',(-28.0251707688815,28.5410196624969,19.));
#46234=CARTESIAN_POINT('',(-28.0251707688815,28.5410196624969,19.));
#46235=CARTESIAN_POINT('Origin',(0.,0.,19.));
#46236=CARTESIAN_POINT('Origin',(0.,0.,19.));
#46237=CARTESIAN_POINT('Origin',(38.7298334620742,10.,19.));
#46238=CARTESIAN_POINT('',(38.7298334620742,10.,19.));
#46239=CARTESIAN_POINT('Origin',(-10.7046626931927,-38.5410196624968,19.));
#46240=CARTESIAN_POINT('',(-10.7046626931927,-38.5410196624968,19.));
#46241=CARTESIAN_POINT('Origin',(5.98741461555926,0.,19.));
#75322=UNCERTAINTY_MEASURE_WITH_UNIT(LENGTH_MEASURE(0.01),#75337,
'DISTANCE_ACCURACY_VALUE',
'Maximum model space distance between geometric entities at asserted c
onnectivities');
#75326=UNCERTAINTY_MEASURE_WITH_UNIT(LENGTH_MEASURE(0.01),#75337,
'DISTANCE_ACCURACY_VALUE',
'Maximum model space distance between geometric entities at asserted c
onnectivities');
#75332=(
GEOMETRIC_REPRESENTATION_CONTEXT(3)
GLOBAL_UNCERTAINTY_ASSIGNED_CONTEXT((#75322))
GLOBAL_UNIT_ASSIGNED_CONTEXT((#75337,#75339,#75340))
REPRESENTATION_CONTEXT('','3D')
);
#75336=(
GEOMETRIC_REPRESENTATION_CONTEXT(3)
GLOBAL_UNCERTAINTY_ASSIGNED_CONTEXT((#75326))
GLOBAL_UNIT_ASSIGNED_CONTEXT((#75337,#75339,#75340))
REPRESENTATION_CONTEXT('','3D')
);
#75337=(
LENGTH_UNIT()
NAMED_UNIT(*)
SI_UNIT(.MILLI.,.METRE.)
);
#75339=(
NAMED_UNIT(*)
PLANE_ANGLE_UNIT()
SI_UNIT($,.RADIAN.)
);
#75340=(
NAMED_UNIT(*)
SI_UNIT($,.STERADIAN.)
SOLID_ANGLE_UNIT()
);
#75346=SHAPE_DEFINITION_REPRESENTATION(#75355,#75372);
#75355=PRODUCT_DEFINITION_SHAPE('',$,#75382);
#75372=SHAPE_REPRESENTATION('',(#32143),#75332);
#75376=PRODUCT_DEFINITION_CONTEXT('part definition',#75405,'design');
#75382=PRODUCT_DEFINITION('Top_Part','Top_Part',#75391,#75376);
#75391=PRODUCT_DEFINITION_FORMATION('',$,#75412);
#75405=APPLICATION_CONTEXT(
'Core Data for Automotive Mechanical Design Process');
#75406=PRODUCT_CONTEXT('part definition',#75405,'mechanical');
#75412=PRODUCT('Top_Part','Top_Part',$,(#75406));
#75417=PRESENTATION_STYLE_ASSIGNMENT((#75421));
#75421=SURFACE_STYLE_USAGE(.BOTH.,#75425);
#75425=SURFACE_SIDE_STYLE('',(#75429));
#75429=SURFACE_STYLE_FILL_AREA(#75433);
#75433=FILL_AREA_STYLE('Opaque(203,203,203)',(#75437));
#75437=FILL_AREA_STYLE_COLOUR('Opaque(203,203,203)',#75441);
#75441=COLOUR_RGB('Opaque(203,203,203)', 0.09019608, 0.27058824, 0.51372549);
ENDSEC;
END-ISO-10303-21;
